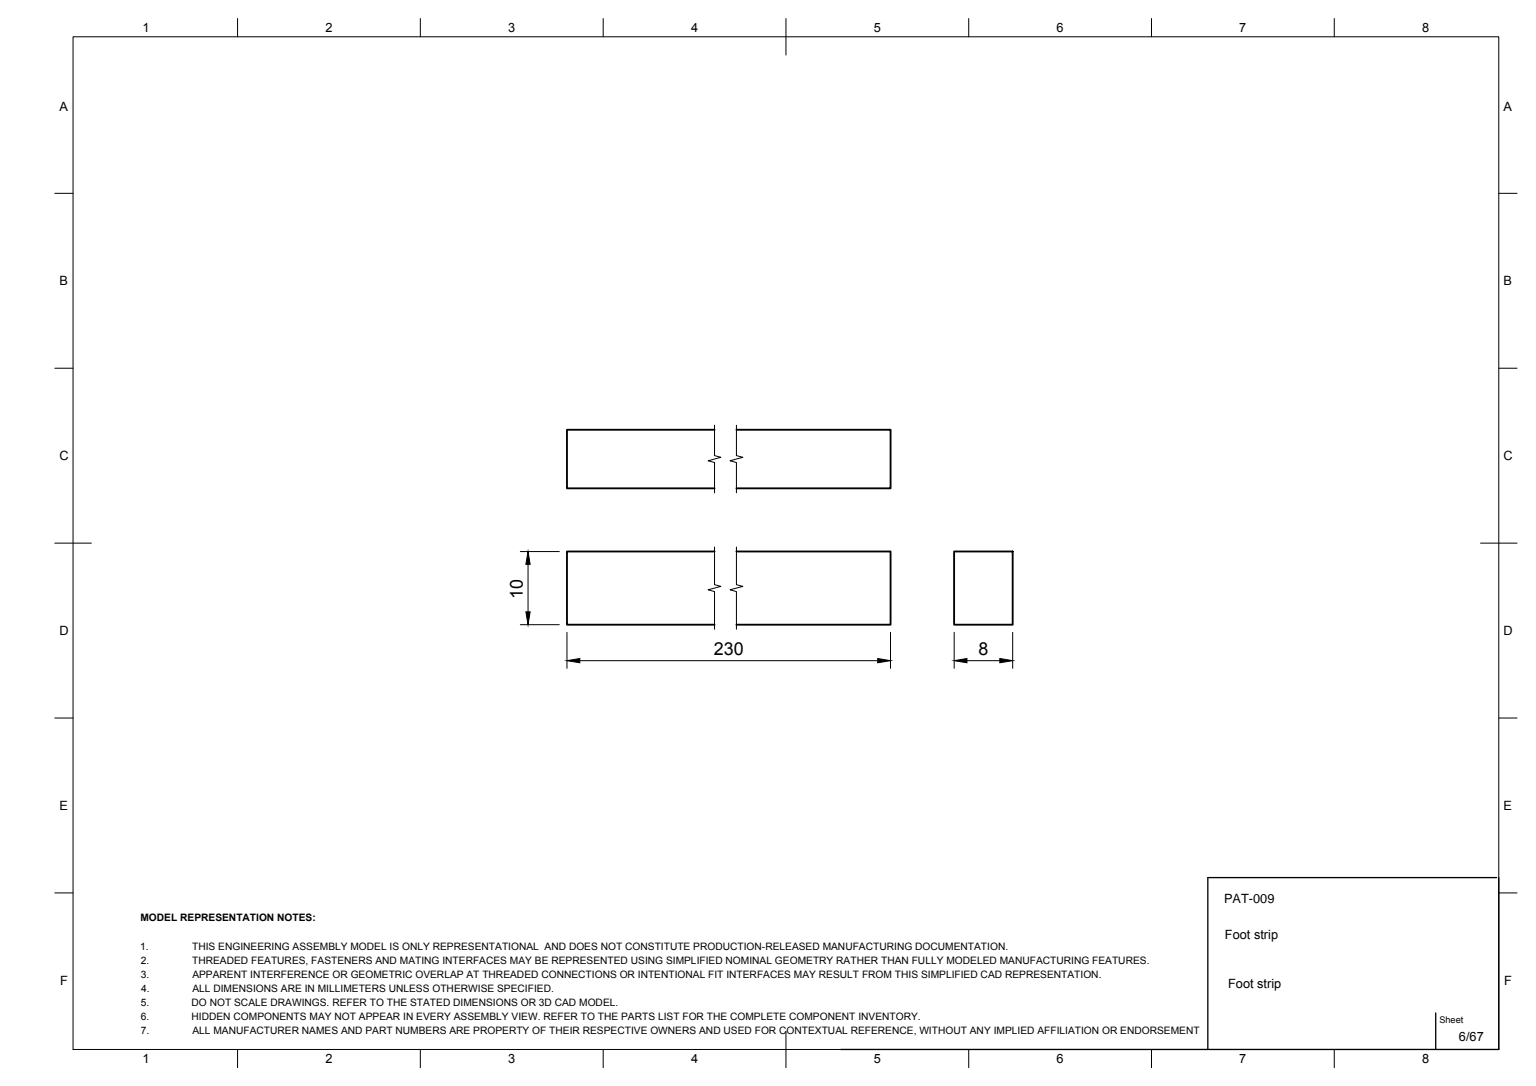
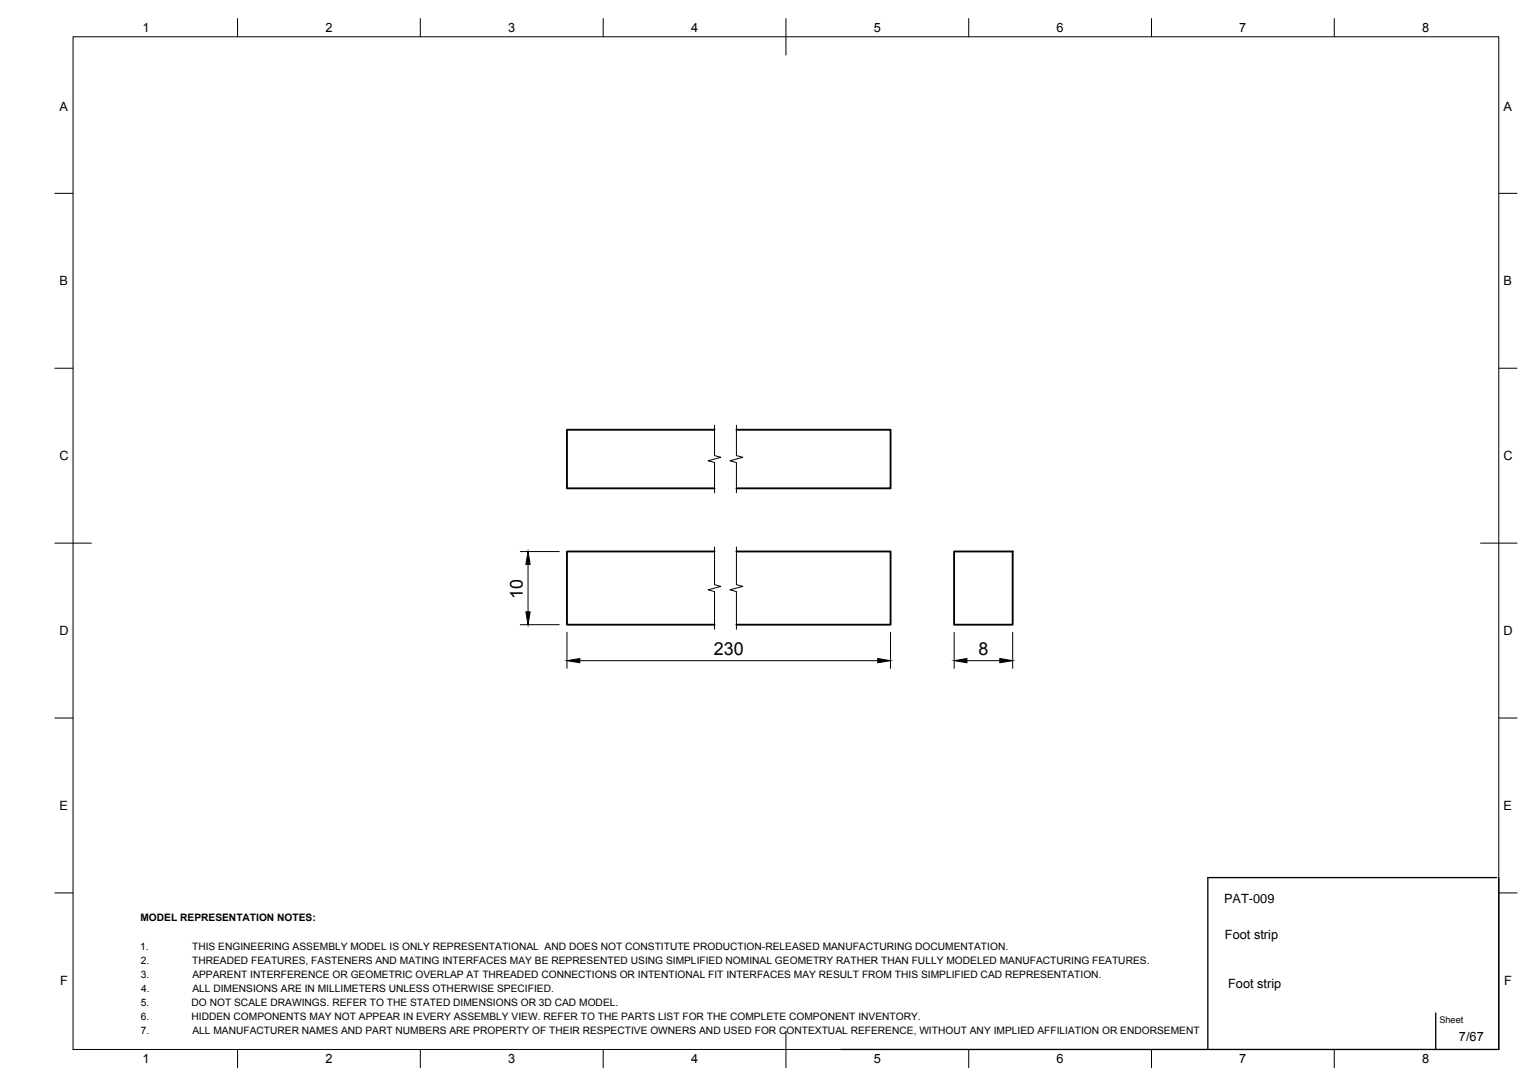
ISO-10303-21;
HEADER;
/* Generated by software containing ST-Developer
 * from STEP Tools, Inc. (www.steptools.com) 
 */

FILE_DESCRIPTION(
/* description */ ('Bell-crank linkage with push rods'),
/* implementation_level */ '2;1');

FILE_NAME(
/* name */ 'Foot strip.step',
/* time_stamp */ '2026-10-28T03:25:15-07:00',
/* author */ (''),
/* organization */ (''),
/* preprocessor_version */ 'ST-DEVELOPER v20.2',
/* originating_system */ 'Autodesk Translation Framework v15.17.0.0',
/* authorisation */ '');

FILE_SCHEMA (('AUTOMOTIVE_DESIGN { 1 0 10303 214 3 1 1 }'));
ENDSEC;

DATA;
#10=MECHANICAL_DESIGN_GEOMETRIC_PRESENTATION_REPRESENTATION('',(#605),#16678);
#497=SHAPE_REPRESENTATION_RELATIONSHIP('SRR','None',#16913,#551);
#551=ADVANCED_BREP_SHAPE_REPRESENTATION('',(#667),#16618);
#605=STYLED_ITEM('',(#17277),#667);
#667=MANIFOLD_SOLID_BREP('Body1',#8795);
#972=PLANE('',#9500);
#973=PLANE('',#9501);
#974=PLANE('',#9502);
#975=PLANE('',#9503);
#976=PLANE('',#9504);
#977=PLANE('',#9505);
#1265=FACE_OUTER_BOUND('',#1811,.T.);
#1266=FACE_OUTER_BOUND('',#1812,.T.);
#1267=FACE_OUTER_BOUND('',#1813,.T.);
#1268=FACE_OUTER_BOUND('',#1814,.T.);
#1269=FACE_OUTER_BOUND('',#1815,.T.);
#1270=FACE_OUTER_BOUND('',#1816,.T.);
#1811=EDGE_LOOP('',(#6007,#6008,#6009,#6010));
#1812=EDGE_LOOP('',(#6011,#6012,#6013,#6014));
#1813=EDGE_LOOP('',(#6015,#6016,#6017,#6018));
#1814=EDGE_LOOP('',(#6019,#6020,#6021,#6022));
#1815=EDGE_LOOP('',(#6023,#6024,#6025,#6026));
#1816=EDGE_LOOP('',(#6027,#6028,#6029,#6030));
#2556=LINE('',#13636,#3105);
#2557=LINE('',#13638,#3106);
#2558=LINE('',#13640,#3107);
#2559=LINE('',#13641,#3108);
#2560=LINE('',#13644,#3109);
#2561=LINE('',#13646,#3110);
#2562=LINE('',#13647,#3111);
#2563=LINE('',#13650,#3112);
#2564=LINE('',#13652,#3113);
#2565=LINE('',#13653,#3114);
#2566=LINE('',#13655,#3115);
#2567=LINE('',#13656,#3116);
#3105=VECTOR('',#10748,1.);
#3106=VECTOR('',#10749,1.);
#3107=VECTOR('',#10750,1.);
#3108=VECTOR('',#10751,1.);
#3109=VECTOR('',#10754,1.);
#3110=VECTOR('',#10755,1.);
#3111=VECTOR('',#10756,1.);
#3112=VECTOR('',#10759,1.);
#3113=VECTOR('',#10760,1.);
#3114=VECTOR('',#10761,1.);
#3115=VECTOR('',#10764,1.);
#3116=VECTOR('',#10765,1.);
#4152=VERTEX_POINT('',#13634);
#4153=VERTEX_POINT('',#13635);
#4154=VERTEX_POINT('',#13637);
#4155=VERTEX_POINT('',#13639);
#4156=VERTEX_POINT('',#13643);
#4157=VERTEX_POINT('',#13645);
#4158=VERTEX_POINT('',#13649);
#4159=VERTEX_POINT('',#13651);
#4881=EDGE_CURVE('',#4152,#4153,#2556,.T.);
#4882=EDGE_CURVE('',#4153,#4154,#2557,.T.);
#4883=EDGE_CURVE('',#4155,#4154,#2558,.T.);
#4884=EDGE_CURVE('',#4152,#4155,#2559,.T.);
#4885=EDGE_CURVE('',#4156,#4152,#2560,.T.);
#4886=EDGE_CURVE('',#4157,#4155,#2561,.T.);
#4887=EDGE_CURVE('',#4156,#4157,#2562,.T.);
#4888=EDGE_CURVE('',#4158,#4156,#2563,.T.);
#4889=EDGE_CURVE('',#4159,#4157,#2564,.T.);
#4890=EDGE_CURVE('',#4158,#4159,#2565,.T.);
#4891=EDGE_CURVE('',#4153,#4158,#2566,.T.);
#4892=EDGE_CURVE('',#4154,#4159,#2567,.T.);
#6007=ORIENTED_EDGE('',*,*,#4881,.T.);
#6008=ORIENTED_EDGE('',*,*,#4882,.T.);
#6009=ORIENTED_EDGE('',*,*,#4883,.F.);
#6010=ORIENTED_EDGE('',*,*,#4884,.F.);
#6011=ORIENTED_EDGE('',*,*,#4885,.T.);
#6012=ORIENTED_EDGE('',*,*,#4884,.T.);
#6013=ORIENTED_EDGE('',*,*,#4886,.F.);
#6014=ORIENTED_EDGE('',*,*,#4887,.F.);
#6015=ORIENTED_EDGE('',*,*,#4888,.T.);
#6016=ORIENTED_EDGE('',*,*,#4887,.T.);
#6017=ORIENTED_EDGE('',*,*,#4889,.F.);
#6018=ORIENTED_EDGE('',*,*,#4890,.F.);
#6019=ORIENTED_EDGE('',*,*,#4891,.T.);
#6020=ORIENTED_EDGE('',*,*,#4890,.T.);
#6021=ORIENTED_EDGE('',*,*,#4892,.F.);
#6022=ORIENTED_EDGE('',*,*,#4882,.F.);
#6023=ORIENTED_EDGE('',*,*,#4892,.T.);
#6024=ORIENTED_EDGE('',*,*,#4889,.T.);
#6025=ORIENTED_EDGE('',*,*,#4886,.T.);
#6026=ORIENTED_EDGE('',*,*,#4883,.T.);
#6027=ORIENTED_EDGE('',*,*,#4891,.F.);
#6028=ORIENTED_EDGE('',*,*,#4881,.F.);
#6029=ORIENTED_EDGE('',*,*,#4885,.F.);
#6030=ORIENTED_EDGE('',*,*,#4888,.F.);
#8290=ADVANCED_FACE('',(#1265),#972,.T.);
#8291=ADVANCED_FACE('',(#1266),#973,.T.);
#8292=ADVANCED_FACE('',(#1267),#974,.T.);
#8293=ADVANCED_FACE('',(#1268),#975,.T.);
#8294=ADVANCED_FACE('',(#1269),#976,.T.);
#8295=ADVANCED_FACE('',(#1270),#977,.F.);
#8795=CLOSED_SHELL('',(#8290,#8291,#8292,#8293,#8294,#8295));
#9499=AXIS2_PLACEMENT_3D('',#13632,#10744,#10745);
#9500=AXIS2_PLACEMENT_3D('',#13633,#10746,#10747);
#9501=AXIS2_PLACEMENT_3D('',#13642,#10752,#10753);
#9502=AXIS2_PLACEMENT_3D('',#13648,#10757,#10758);
#9503=AXIS2_PLACEMENT_3D('',#13654,#10762,#10763);
#9504=AXIS2_PLACEMENT_3D('',#13657,#10766,#10767);
#9505=AXIS2_PLACEMENT_3D('',#13658,#10768,#10769);
#10744=DIRECTION('axis',(0.,0.,1.));
#10745=DIRECTION('refdir',(1.,0.,0.));
#10746=DIRECTION('center_axis',(0.,1.,0.));
#10747=DIRECTION('ref_axis',(-1.,0.,0.));
#10748=DIRECTION('',(-1.,0.,0.));
#10749=DIRECTION('',(0.,0.,1.));
#10750=DIRECTION('',(-1.,0.,0.));
#10751=DIRECTION('',(0.,0.,1.));
#10752=DIRECTION('center_axis',(1.,0.,0.));
#10753=DIRECTION('ref_axis',(0.,1.,0.));
#10754=DIRECTION('',(0.,1.,0.));
#10755=DIRECTION('',(0.,1.,0.));
#10756=DIRECTION('',(0.,0.,1.));
#10757=DIRECTION('center_axis',(0.,-1.,0.));
#10758=DIRECTION('ref_axis',(1.,0.,0.));
#10759=DIRECTION('',(1.,0.,0.));
#10760=DIRECTION('',(1.,0.,0.));
#10761=DIRECTION('',(0.,0.,1.));
#10762=DIRECTION('center_axis',(-1.,0.,0.));
#10763=DIRECTION('ref_axis',(0.,-1.,0.));
#10764=DIRECTION('',(0.,-1.,0.));
#10765=DIRECTION('',(0.,-1.,0.));
#10766=DIRECTION('center_axis',(0.,0.,1.));
#10767=DIRECTION('ref_axis',(1.,0.,0.));
#10768=DIRECTION('center_axis',(0.,0.,1.));
#10769=DIRECTION('ref_axis',(1.,0.,0.));
#13632=CARTESIAN_POINT('',(0.,0.,0.));
#13633=CARTESIAN_POINT('Origin',(-3.,19.,-0.8));
#13634=CARTESIAN_POINT('',(-3.,19.,-0.8));
#13635=CARTESIAN_POINT('',(-4.,19.,-0.8));
#13636=CARTESIAN_POINT('',(-3.,19.,-0.8));
#13637=CARTESIAN_POINT('',(-4.,19.,0.));
#13638=CARTESIAN_POINT('',(-4.,19.,-0.8));
#13639=CARTESIAN_POINT('',(-3.,19.,0.));
#13640=CARTESIAN_POINT('',(-3.,19.,0.));
#13641=CARTESIAN_POINT('',(-3.,19.,-0.8));
#13642=CARTESIAN_POINT('Origin',(-3.,-4.,-0.8));
#13643=CARTESIAN_POINT('',(-3.,-4.,-0.8));
#13644=CARTESIAN_POINT('',(-3.,-4.,-0.8));
#13645=CARTESIAN_POINT('',(-3.,-4.,0.));
#13646=CARTESIAN_POINT('',(-3.,-4.,0.));
#13647=CARTESIAN_POINT('',(-3.,-4.,-0.8));
#13648=CARTESIAN_POINT('Origin',(-4.,-4.,-0.8));
#13649=CARTESIAN_POINT('',(-4.,-4.,-0.8));
#13650=CARTESIAN_POINT('',(-4.,-4.,-0.8));
#13651=CARTESIAN_POINT('',(-4.,-4.,0.));
#13652=CARTESIAN_POINT('',(-4.,-4.,0.));
#13653=CARTESIAN_POINT('',(-4.,-4.,-0.8));
#13654=CARTESIAN_POINT('Origin',(-4.,19.,-0.8));
#13655=CARTESIAN_POINT('',(-4.,19.,-0.8));
#13656=CARTESIAN_POINT('',(-4.,19.,0.));
#13657=CARTESIAN_POINT('Origin',(-3.5,7.5,0.));
#13658=CARTESIAN_POINT('Origin',(-3.5,7.5,-0.8));
#16554=UNCERTAINTY_MEASURE_WITH_UNIT(LENGTH_MEASURE(0.001),#16679,
'DISTANCE_ACCURACY_VALUE',
'Maximum model space distance between geometric entities at asserted c
onnectivities');
#16614=UNCERTAINTY_MEASURE_WITH_UNIT(LENGTH_MEASURE(0.001),#16679,
'DISTANCE_ACCURACY_VALUE',
'Maximum model space distance between geometric entities at asserted c
onnectivities');
#16618=(
GEOMETRIC_REPRESENTATION_CONTEXT(3)
GLOBAL_UNCERTAINTY_ASSIGNED_CONTEXT((#16554))
GLOBAL_UNIT_ASSIGNED_CONTEXT((#16679,#16681,#16682))
REPRESENTATION_CONTEXT('','3D')
);
#16678=(
GEOMETRIC_REPRESENTATION_CONTEXT(3)
GLOBAL_UNCERTAINTY_ASSIGNED_CONTEXT((#16614))
GLOBAL_UNIT_ASSIGNED_CONTEXT((#16679,#16681,#16682))
REPRESENTATION_CONTEXT('','3D')
);
#16679=(
LENGTH_UNIT()
NAMED_UNIT(*)
SI_UNIT(.CENTI.,.METRE.)
);
#16681=(
NAMED_UNIT(*)
PLANE_ANGLE_UNIT()
SI_UNIT($,.RADIAN.)
);
#16682=(
NAMED_UNIT(*)
SI_UNIT($,.STERADIAN.)
SOLID_ANGLE_UNIT()
);
#16686=SHAPE_DEFINITION_REPRESENTATION(#16749,#16913);
#16749=PRODUCT_DEFINITION_SHAPE('',$,#16977);
#16913=SHAPE_REPRESENTATION('',(#9499),#16618);
#16973=PRODUCT_DEFINITION_CONTEXT('part definition',#17164,'design');
#16977=PRODUCT_DEFINITION('Foot strip','Foot strip',#17040,#16973);
#17040=PRODUCT_DEFINITION_FORMATION('',$,#17169);
#17164=APPLICATION_CONTEXT(
'Core Data for Automotive Mechanical Design Process');
#17165=PRODUCT_CONTEXT('part definition',#17164,'mechanical');
#17169=PRODUCT('Foot strip','Foot strip','Foot strip',(#17165));
#17271=COLOUR_RGB('Light Blue',0.38,0.62,0.78);
#17272=FILL_AREA_STYLE_COLOUR('',#17271);
#17273=FILL_AREA_STYLE('',(#17272));
#17274=SURFACE_STYLE_FILL_AREA(#17273);
#17275=SURFACE_SIDE_STYLE('',(#17274));
#17276=SURFACE_STYLE_USAGE(.BOTH.,#17275);
#17277=PRESENTATION_STYLE_ASSIGNMENT((#17276));
ENDSEC;
END-ISO-10303-21;
